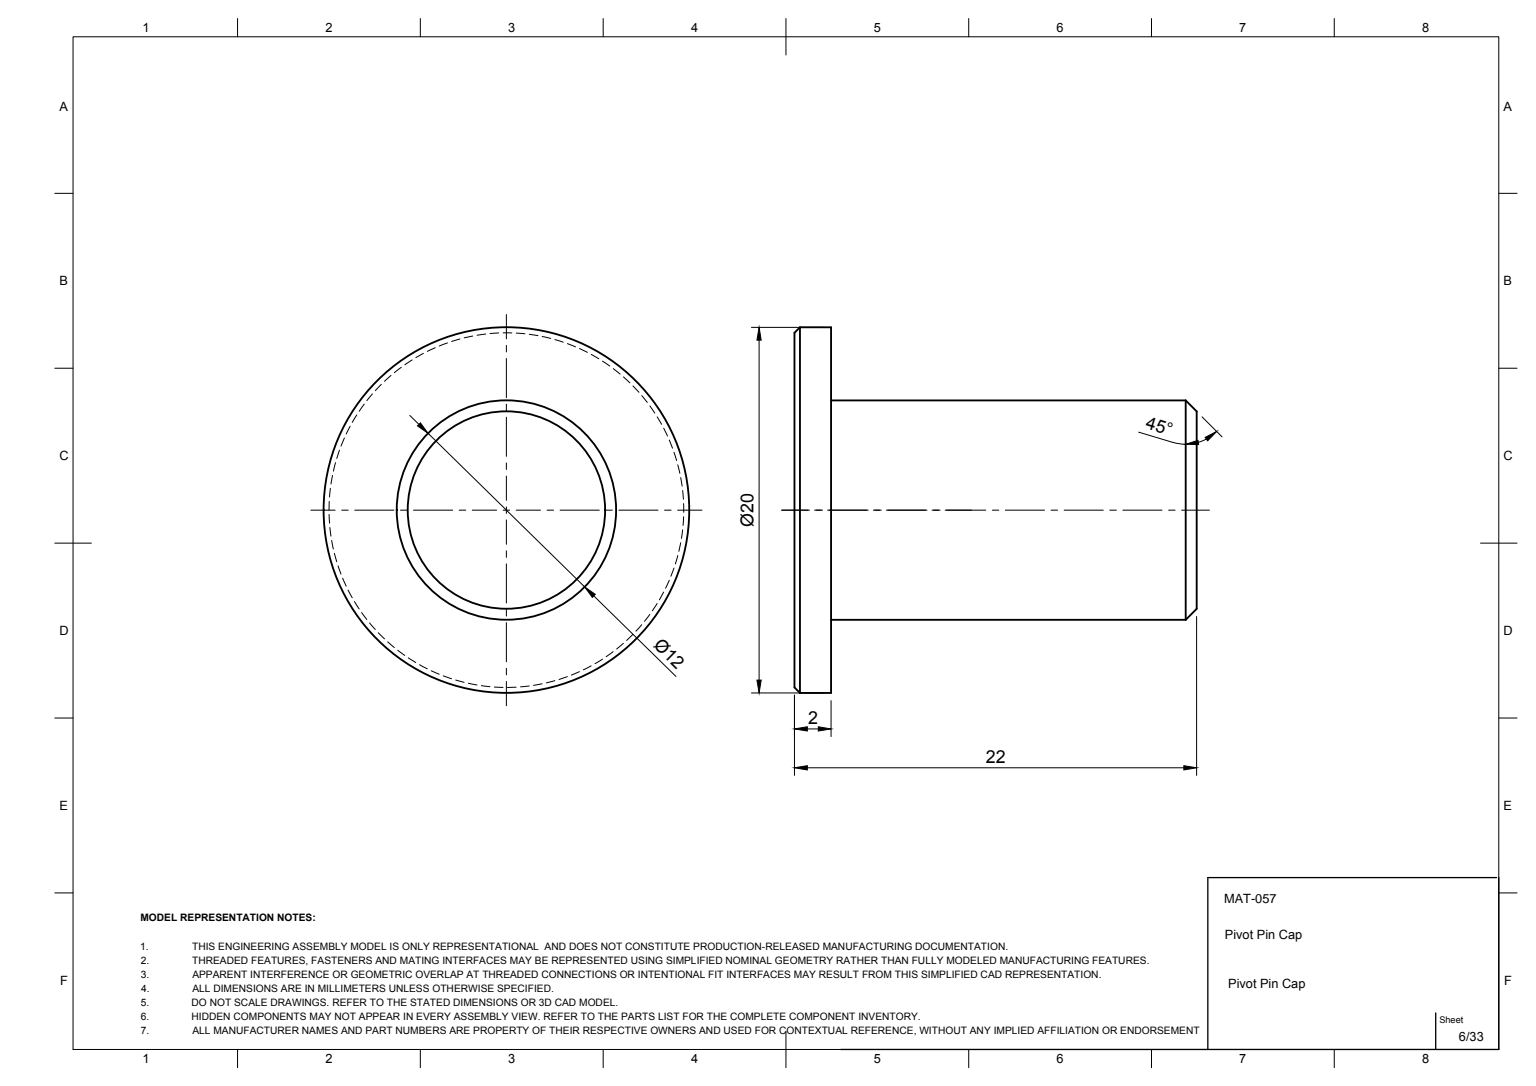
ISO-10303-21;
HEADER;
/* Generated by software containing ST-Developer
 * from STEP Tools, Inc. (www.steptools.com) 
 */

FILE_DESCRIPTION(
/* description */ ('STEP AP214', 'CAx-IF Rec.Pracs.---Representation and Presentation of Product Manufa
cturing Information (PMI)---4.0---2014-10-13'),
/* implementation_level */ '2;1');

FILE_NAME(
/* name */ 'Pivot Pin Cap.step',
/* time_stamp */ '2026-10-28T23:34:22+01:00',
/* author */ (''),
/* organization */ (''),
/* preprocessor_version */ 'ST-DEVELOPER v20.2',
/* originating_system */ 'Autodesk Translation Framework v15.17.0.0',
/* authorisation */ '');

FILE_SCHEMA (('AP242_MANAGED_MODEL_BASED_3D_ENGINEERING_MIM_LF { 1 0 10303 442 2 1 4 }'));
ENDSEC;

DATA;
#10=MECHANICAL_DESIGN_GEOMETRIC_PRESENTATION_REPRESENTATION('',(#277),#27807);
#226=SHAPE_REPRESENTATION_RELATIONSHIP('SRR','None',#27925,#248);
#248=ADVANCED_BREP_SHAPE_REPRESENTATION('',(#306),#27805);
#277=STYLED_ITEM('',(#28077),#306);
#306=MANIFOLD_SOLID_BREP('Body1',#12053);
#447=FACE_BOUND('',#2748,.T.);
#742=PLANE('',#13705);
#743=PLANE('',#13706);
#744=PLANE('',#13707);
#1244=CYLINDRICAL_SURFACE('',#13701,10.);
#1245=CYLINDRICAL_SURFACE('',#13703,6.);
#1932=FACE_OUTER_BOUND('',#2741,.T.);
#1933=FACE_OUTER_BOUND('',#2742,.T.);
#1934=FACE_OUTER_BOUND('',#2743,.T.);
#1935=FACE_OUTER_BOUND('',#2744,.T.);
#1936=FACE_OUTER_BOUND('',#2745,.T.);
#1937=FACE_OUTER_BOUND('',#2746,.T.);
#1938=FACE_OUTER_BOUND('',#2747,.T.);
#2741=EDGE_LOOP('',(#11239,#11240,#11241,#11242));
#2742=EDGE_LOOP('',(#11243,#11244,#11245,#11246,#11247));
#2743=EDGE_LOOP('',(#11248,#11249,#11250,#11251));
#2744=EDGE_LOOP('',(#11252,#11253,#11254,#11255,#11256));
#2745=EDGE_LOOP('',(#11257));
#2746=EDGE_LOOP('',(#11258));
#2747=EDGE_LOOP('',(#11259));
#2748=EDGE_LOOP('',(#11260));
#3567=LINE('',#27697,#4387);
#3568=LINE('',#27705,#4388);
#3569=LINE('',#27710,#4389);
#3570=LINE('',#27713,#4390);
#4387=VECTOR('',#17341,9.70000000000001);
#4388=VECTOR('',#17350,6.);
#4389=VECTOR('',#17357,10.);
#4390=VECTOR('',#17360,6.);
#5023=CIRCLE('',#13695,10.);
#5024=CIRCLE('',#13696,9.7);
#5025=CIRCLE('',#13698,6.);
#5026=CIRCLE('',#13699,6.);
#5027=CIRCLE('',#13700,5.4);
#5028=CIRCLE('',#13702,10.);
#5029=CIRCLE('',#13704,6.);
#6126=VERTEX_POINT('',#27694);
#6127=VERTEX_POINT('',#27696);
#6128=VERTEX_POINT('',#27700);
#6129=VERTEX_POINT('',#27701);
#6130=VERTEX_POINT('',#27704);
#6131=VERTEX_POINT('',#27708);
#6132=VERTEX_POINT('',#27712);
#7832=EDGE_CURVE('',#6126,#6126,#5023,.T.);
#7833=EDGE_CURVE('',#6126,#6127,#3567,.T.);
#7834=EDGE_CURVE('',#6127,#6127,#5024,.T.);
#7835=EDGE_CURVE('',#6128,#6129,#5025,.T.);
#7836=EDGE_CURVE('',#6129,#6128,#5026,.T.);
#7837=EDGE_CURVE('',#6129,#6130,#3568,.T.);
#7838=EDGE_CURVE('',#6130,#6130,#5027,.T.);
#7839=EDGE_CURVE('',#6131,#6131,#5028,.T.);
#7840=EDGE_CURVE('',#6131,#6126,#3569,.T.);
#7841=EDGE_CURVE('',#6128,#6132,#3570,.T.);
#7842=EDGE_CURVE('',#6132,#6132,#5029,.T.);
#11239=ORIENTED_EDGE('',*,*,#7832,.F.);
#11240=ORIENTED_EDGE('',*,*,#7833,.T.);
#11241=ORIENTED_EDGE('',*,*,#7834,.F.);
#11242=ORIENTED_EDGE('',*,*,#7833,.F.);
#11243=ORIENTED_EDGE('',*,*,#7835,.F.);
#11244=ORIENTED_EDGE('',*,*,#7836,.F.);
#11245=ORIENTED_EDGE('',*,*,#7837,.T.);
#11246=ORIENTED_EDGE('',*,*,#7838,.F.);
#11247=ORIENTED_EDGE('',*,*,#7837,.F.);
#11248=ORIENTED_EDGE('',*,*,#7839,.T.);
#11249=ORIENTED_EDGE('',*,*,#7840,.T.);
#11250=ORIENTED_EDGE('',*,*,#7832,.T.);
#11251=ORIENTED_EDGE('',*,*,#7840,.F.);
#11252=ORIENTED_EDGE('',*,*,#7835,.T.);
#11253=ORIENTED_EDGE('',*,*,#7836,.T.);
#11254=ORIENTED_EDGE('',*,*,#7841,.T.);
#11255=ORIENTED_EDGE('',*,*,#7842,.F.);
#11256=ORIENTED_EDGE('',*,*,#7841,.F.);
#11257=ORIENTED_EDGE('',*,*,#7838,.T.);
#11258=ORIENTED_EDGE('',*,*,#7834,.T.);
#11259=ORIENTED_EDGE('',*,*,#7839,.F.);
#11260=ORIENTED_EDGE('',*,*,#7842,.T.);
#11325=CONICAL_SURFACE('',#13694,9.70000000000001,0.785398163397434);
#11326=CONICAL_SURFACE('',#13697,6.,0.785398163397452);
#12014=ADVANCED_FACE('',(#1932),#11325,.T.);
#12015=ADVANCED_FACE('',(#1933),#11326,.T.);
#12016=ADVANCED_FACE('',(#1934),#1244,.T.);
#12017=ADVANCED_FACE('',(#1935),#1245,.T.);
#12018=ADVANCED_FACE('',(#1936),#742,.F.);
#12019=ADVANCED_FACE('',(#1937),#743,.T.);
#12020=ADVANCED_FACE('',(#1938,#447),#744,.F.);
#12053=CLOSED_SHELL('',(#12014,#12015,#12016,#12017,#12018,#12019,#12020));
#13693=AXIS2_PLACEMENT_3D('',#27692,#17335,#17336);
#13694=AXIS2_PLACEMENT_3D('',#27693,#17337,#17338);
#13695=AXIS2_PLACEMENT_3D('',#27695,#17339,#17340);
#13696=AXIS2_PLACEMENT_3D('',#27698,#17342,#17343);
#13697=AXIS2_PLACEMENT_3D('',#27699,#17344,#17345);
#13698=AXIS2_PLACEMENT_3D('',#27702,#17346,#17347);
#13699=AXIS2_PLACEMENT_3D('',#27703,#17348,#17349);
#13700=AXIS2_PLACEMENT_3D('',#27706,#17351,#17352);
#13701=AXIS2_PLACEMENT_3D('',#27707,#17353,#17354);
#13702=AXIS2_PLACEMENT_3D('',#27709,#17355,#17356);
#13703=AXIS2_PLACEMENT_3D('',#27711,#17358,#17359);
#13704=AXIS2_PLACEMENT_3D('',#27714,#17361,#17362);
#13705=AXIS2_PLACEMENT_3D('',#27715,#17363,#17364);
#13706=AXIS2_PLACEMENT_3D('',#27716,#17365,#17366);
#13707=AXIS2_PLACEMENT_3D('',#27717,#17367,#17368);
#17335=DIRECTION('axis',(0.,0.,1.));
#17336=DIRECTION('refdir',(1.,0.,0.));
#17337=DIRECTION('center_axis',(0.,0.,1.));
#17338=DIRECTION('ref_axis',(0.893719561472763,-0.448626064156924,0.));
#17339=DIRECTION('center_axis',(0.,0.,1.));
#17340=DIRECTION('ref_axis',(-0.893719561472763,0.448626064156923,0.));
#17341=DIRECTION('',(0.631955162396449,-0.317226532182388,-0.707106781186558));
#17342=DIRECTION('center_axis',(0.,0.,-1.));
#17343=DIRECTION('ref_axis',(-0.893719561472763,0.448626064156925,0.));
#17344=DIRECTION('center_axis',(0.,0.,-1.));
#17345=DIRECTION('ref_axis',(-0.893719561472763,0.448626064156923,0.));
#17346=DIRECTION('center_axis',(0.,0.,-1.));
#17347=DIRECTION('ref_axis',(-0.893719561472763,0.448626064156923,0.));
#17348=DIRECTION('center_axis',(0.,0.,-1.));
#17349=DIRECTION('ref_axis',(-0.893719561472763,0.448626064156923,0.));
#17350=DIRECTION('',(-0.631955162396461,0.317226532182393,0.707106781186545));
#17351=DIRECTION('center_axis',(0.,0.,1.));
#17352=DIRECTION('ref_axis',(-0.893719561472762,0.448626064156926,0.));
#17353=DIRECTION('center_axis',(0.,0.,1.));
#17354=DIRECTION('ref_axis',(0.893719561472763,-0.448626064156924,0.));
#17355=DIRECTION('center_axis',(0.,0.,-1.));
#17356=DIRECTION('ref_axis',(-0.893719561472763,0.448626064156923,0.));
#17357=DIRECTION('',(0.,0.,-1.));
#17358=DIRECTION('center_axis',(0.,0.,1.));
#17359=DIRECTION('ref_axis',(0.893719561472763,-0.448626064156923,0.));
#17360=DIRECTION('',(0.,0.,-1.));
#17361=DIRECTION('center_axis',(0.,0.,-1.));
#17362=DIRECTION('ref_axis',(-0.893719561472763,0.448626064156923,0.));
#17363=DIRECTION('center_axis',(0.,0.,-1.));
#17364=DIRECTION('ref_axis',(-0.893719561472763,0.448626064156924,0.));
#17365=DIRECTION('center_axis',(0.,0.,-1.));
#17366=DIRECTION('ref_axis',(-0.893719561472763,0.448626064156924,0.));
#17367=DIRECTION('center_axis',(0.,0.,-1.));
#17368=DIRECTION('ref_axis',(-0.893719561472763,0.448626064156924,0.));
#27692=CARTESIAN_POINT('',(0.,0.,0.));
#27693=CARTESIAN_POINT('Origin',(11.0200923794881,112.698833864687,276.073593133701));
#27694=CARTESIAN_POINT('',(2.0828967647605,117.185094506256,276.373593133701));
#27695=CARTESIAN_POINT('Origin',(11.0200923794881,112.698833864687,276.373593133701));
#27696=CARTESIAN_POINT('',(2.35101263320233,117.050506687009,276.073593133701));
#27697=CARTESIAN_POINT('',(2.35101263320233,117.050506687009,276.073593133701));
#27698=CARTESIAN_POINT('Origin',(11.0200923794881,112.698833864687,276.073593133701));
#27699=CARTESIAN_POINT('Origin',(11.0200923794881,112.698833864687,297.473593133701));
#27700=CARTESIAN_POINT('',(5.65777501065156,115.390590249628,297.473593133701));
#27701=CARTESIAN_POINT('',(16.3824097483247,110.007077479745,297.473593133701));
#27702=CARTESIAN_POINT('Origin',(11.0200923794881,112.698833864687,297.473593133701));
#27703=CARTESIAN_POINT('Origin',(11.0200923794881,112.698833864687,297.473593133701));
#27704=CARTESIAN_POINT('',(15.8461780114411,110.276253118239,298.073593133701));
#27705=CARTESIAN_POINT('',(16.3824097483247,110.007077479745,297.473593133701));
#27706=CARTESIAN_POINT('Origin',(11.0200923794881,112.698833864687,298.073593133701));
#27707=CARTESIAN_POINT('Origin',(11.0200923794881,112.698833864687,276.073593133701));
#27708=CARTESIAN_POINT('',(2.0828967647605,117.185094506256,278.073593133701));
#27709=CARTESIAN_POINT('Origin',(11.0200923794881,112.698833864687,278.073593133701));
#27710=CARTESIAN_POINT('',(2.0828967647605,117.185094506256,276.073593133701));
#27711=CARTESIAN_POINT('Origin',(11.0200923794881,112.698833864687,278.073593133701));
#27712=CARTESIAN_POINT('',(5.65777501065155,115.390590249628,278.073593133701));
#27713=CARTESIAN_POINT('',(5.65777501065155,115.390590249628,278.073593133701));
#27714=CARTESIAN_POINT('Origin',(11.0200923794881,112.698833864687,278.073593133701));
#27715=CARTESIAN_POINT('Origin',(11.0200923794881,112.698833864687,298.073593133701));
#27716=CARTESIAN_POINT('Origin',(11.0200923794881,112.698833864687,276.073593133701));
#27717=CARTESIAN_POINT('Origin',(11.0200923794881,112.698833864687,278.073593133701));
#27776=UNCERTAINTY_MEASURE_WITH_UNIT(LENGTH_MEASURE(0.01),#27808,
'DISTANCE_ACCURACY_VALUE',
'Maximum model space distance between geometric entities at asserted c
onnectivities');
#27778=UNCERTAINTY_MEASURE_WITH_UNIT(LENGTH_MEASURE(0.01),#27808,
'DISTANCE_ACCURACY_VALUE',
'Maximum model space distance between geometric entities at asserted c
onnectivities');
#27805=(
GEOMETRIC_REPRESENTATION_CONTEXT(3)
GLOBAL_UNCERTAINTY_ASSIGNED_CONTEXT((#27776))
GLOBAL_UNIT_ASSIGNED_CONTEXT((#27808,#27810,#27811))
REPRESENTATION_CONTEXT('','3D')
);
#27807=(
GEOMETRIC_REPRESENTATION_CONTEXT(3)
GLOBAL_UNCERTAINTY_ASSIGNED_CONTEXT((#27778))
GLOBAL_UNIT_ASSIGNED_CONTEXT((#27808,#27810,#27811))
REPRESENTATION_CONTEXT('','3D')
);
#27808=(
LENGTH_UNIT()
NAMED_UNIT(*)
SI_UNIT(.MILLI.,.METRE.)
);
#27810=(
NAMED_UNIT(*)
PLANE_ANGLE_UNIT()
SI_UNIT($,.RADIAN.)
);
#27811=(
NAMED_UNIT(*)
SI_UNIT($,.STERADIAN.)
SOLID_ANGLE_UNIT()
);
#27838=SHAPE_DEFINITION_REPRESENTATION(#27884,#27925);
#27884=PRODUCT_DEFINITION_SHAPE('',$,#27954);
#27925=SHAPE_REPRESENTATION('',(#13693),#27805);
#27927=PRODUCT_DEFINITION_CONTEXT('part definition',#28013,'design');
#27954=PRODUCT_DEFINITION('Pivot Pin Cap','Pivot Pin Cap',#27982,#27927);
#27982=PRODUCT_DEFINITION_FORMATION('',$,#28041);
#28013=APPLICATION_CONTEXT('Managed model based 3d engineering');
#28014=PRODUCT_CONTEXT('part definition',#28013,'mechanical');
#28041=PRODUCT('Pivot Pin Cap','Pivot Pin Cap',$,(#28014));
#28071=COLOUR_RGB('Grey',0.48,0.52,0.57);
#28072=FILL_AREA_STYLE_COLOUR('',#28071);
#28073=FILL_AREA_STYLE('',(#28072));
#28074=SURFACE_STYLE_FILL_AREA(#28073);
#28075=SURFACE_SIDE_STYLE('',(#28074));
#28076=SURFACE_STYLE_USAGE(.BOTH.,#28075);
#28077=PRESENTATION_STYLE_ASSIGNMENT((#28076));
ENDSEC;
END-ISO-10303-21;
